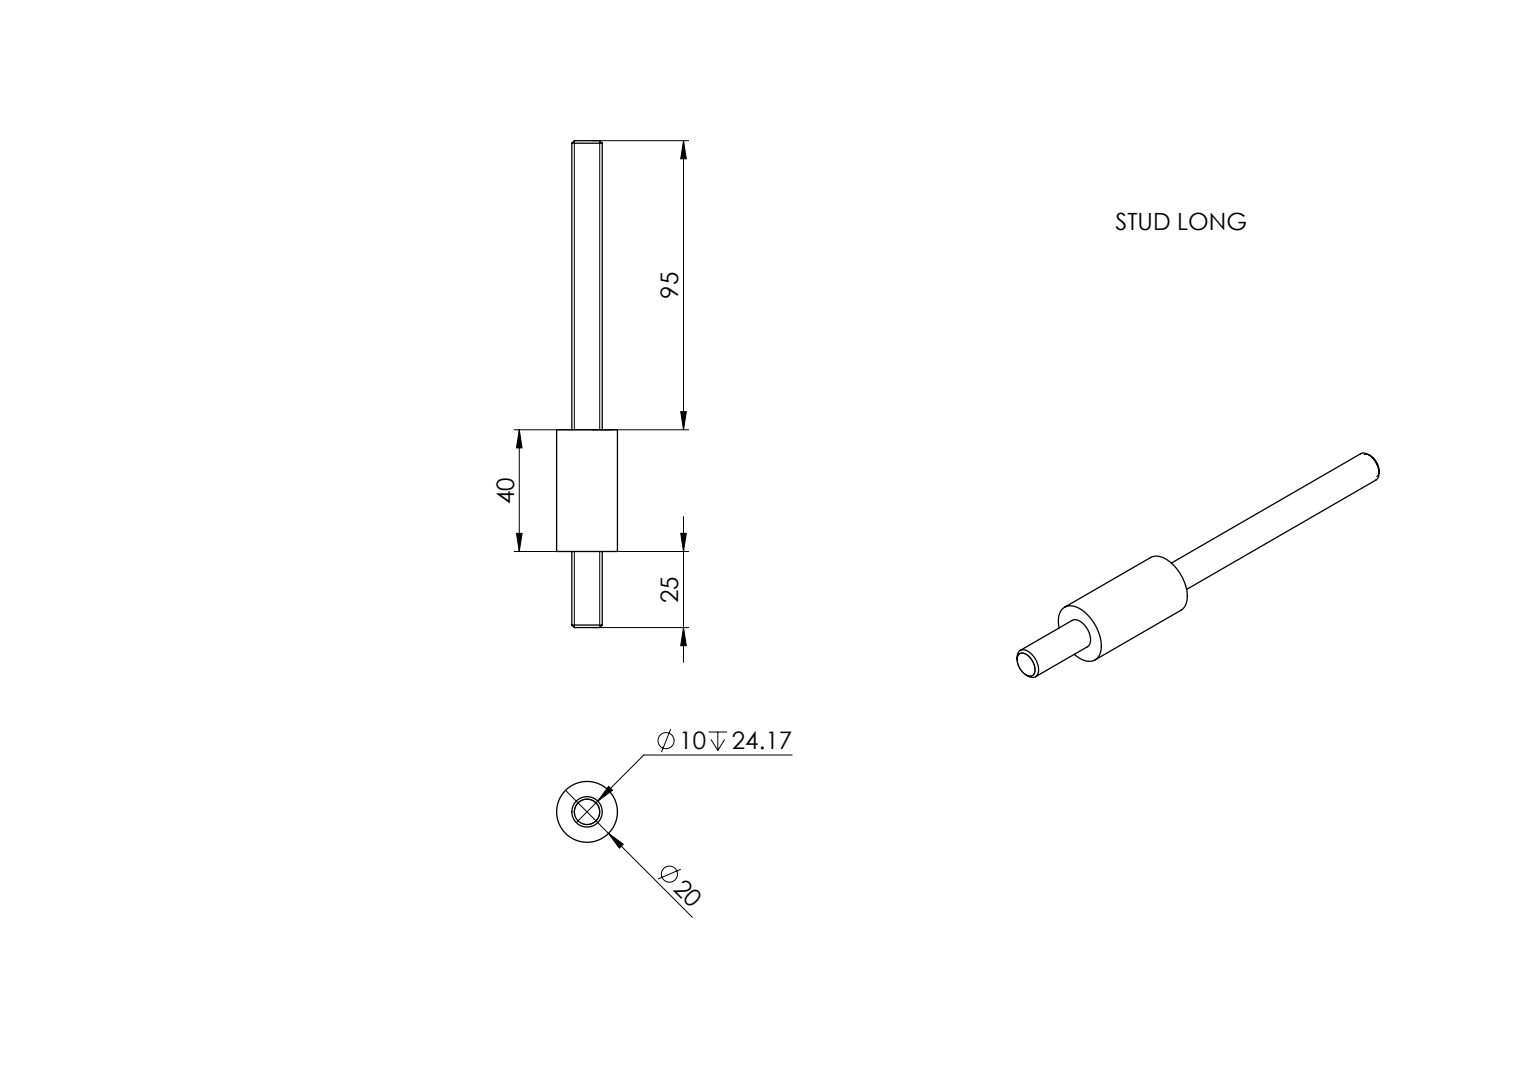
ISO-10303-21;
HEADER;
FILE_DESCRIPTION (('STEP AP214'),
    '1' );
FILE_NAME ('stud long.step',
    '2026-10-23T05:12:30',
    ( '' ),
    ( '' ),
    'SwSTEP 2.0',
    'SolidWorks 2026',
    '' );
FILE_SCHEMA (( 'AUTOMOTIVE_DESIGN' ));
ENDSEC;

DATA;
#5=CARTESIAN_POINT ( 'NONE',  ( -63.76644452187071721, 49.96174644486006855, -40.00000000000000000 ) ) ;
#28=CARTESIAN_POINT ( 'NONE',  ( -58.76644452187068168, 49.96174644486002592, -40.00000000000000000 ) ) ;
#77=DIRECTION ( 'NONE',  ( -0.000000000000000000, -0.000000000000000000, 1.000000000000000000 ) ) ;
#101=DIRECTION ( 'NONE',  ( 0.000000000000000000, 0.000000000000000000, 1.000000000000000000 ) ) ;
#189=CYLINDRICAL_SURFACE ( 'NONE', #7328, 5.000000000000004441 ) ;
#212=DIRECTION ( 'NONE',  ( -0.000000000000000000, -0.000000000000000000, -1.000000000000000000 ) ) ;
#233=DIRECTION ( 'NONE',  ( -1.000000000000000000, 0.000000000000000000, 0.000000000000000000 ) ) ;
#243=LINE ( 'NONE', #4981, #3185 ) ;
#258=AXIS2_PLACEMENT_3D ( 'NONE', #3304, #337, #5703 ) ;
#262=CARTESIAN_POINT ( 'NONE',  ( -68.76644452187068168, 49.96174644486002592, 0.000000000000000000 ) ) ;
#282=CARTESIAN_POINT ( 'NONE',  ( -72.93844452187067873, 49.96174644486002592, 25.00000000000000000 ) ) ;
#290=AXIS2_PLACEMENT_3D ( 'NONE', #4924, #77, #3632 ) ;
#297=AXIS2_PLACEMENT_3D ( 'NONE', #3501, #3421, #499 ) ;
#302=PRODUCT_DEFINITION ( 'UNKNOWN', '', #6087, #1721 ) ;
#312=EDGE_CURVE ( 'NONE', #3677, #520, #3029, .T. ) ;
#316=EDGE_CURVE ( 'NONE', #3677, #1170, #2354, .T. ) ;
#318=CARTESIAN_POINT ( 'NONE',  ( -68.76644452187068168, 49.96174644486002592, 24.17200000000001125 ) ) ;
#320=CARTESIAN_POINT ( 'NONE',  ( -68.76644452187068168, 49.96174644486002592, 24.17200000000001125 ) ) ;
#337=DIRECTION ( 'NONE',  ( 0.000000000000000000, 0.000000000000000000, 1.000000000000000000 ) ) ;
#350=ORIENTED_EDGE ( 'NONE', *, *, #2657, .F. ) ;
#374=EDGE_LOOP ( 'NONE', ( #679, #6781, #2050, #5404 ) ) ;
#380=VERTEX_POINT ( 'NONE', #1396 ) ;
#392=CIRCLE ( 'NONE', #1408, 10.00000000000000178 ) ;
#409=ADVANCED_FACE ( 'NONE', ( #5620 ), #3809, .T. ) ;
#429=STYLED_ITEM('',(#7837),#5821);
#440=ORIENTED_EDGE ( 'NONE', *, *, #2302, .F. ) ;
#455=CARTESIAN_POINT ( 'NONE',  ( -68.76644452187068168, 49.96174644486002592, 0.000000000000000000 ) ) ;
#469=DIRECTION ( 'NONE',  ( 1.000000000000000000, 0.000000000000000000, 0.000000000000000000 ) ) ;
#499=DIRECTION ( 'NONE',  ( 1.000000000000000000, 0.000000000000000000, 0.000000000000000000 ) ) ;
#509=CARTESIAN_POINT ( 'NONE',  ( -68.76644452187072432, 49.96174644486006855, -134.1720000000000255 ) ) ;
#520=VERTEX_POINT ( 'NONE', #2940 ) ;
#533=ORIENTED_EDGE ( 'NONE', *, *, #7554, .T. ) ;
#550=AXIS2_PLACEMENT_3D ( 'NONE', #3748, #3669, #5598 ) ;
#553=EDGE_LOOP ( 'NONE', ( #2394, #4192, #566, #4577 ) ) ;
#561=ORIENTED_EDGE ( 'NONE', *, *, #5713, .F. ) ;
#566=ORIENTED_EDGE ( 'NONE', *, *, #3757, .F. ) ;
#574=( GEOMETRIC_REPRESENTATION_CONTEXT ( 3 ) GLOBAL_UNCERTAINTY_ASSIGNED_CONTEXT ( ( #5327 ) ) GLOBAL_UNIT_ASSIGNED_CONTEXT ( ( #4488, #1529, #2096 ) ) REPRESENTATION_CONTEXT ( 'NONE', 'WORKASPACE' ) );
#581=PLANE ( 'NONE',  #2500 ) ;
#679=ORIENTED_EDGE ( 'NONE', *, *, #312, .F. ) ;
#732=CARTESIAN_POINT ( 'NONE',  ( -63.76644452187073142, 49.96174644486006855, -134.1720000000000255 ) ) ;
#748=CARTESIAN_POINT ( 'NONE',  ( -64.59444452187072727, 49.96174644486006855, -135.0000000000000000 ) ) ;
#810=DIRECTION ( 'NONE',  ( 0.000000000000000000, 0.000000000000000000, 1.000000000000000000 ) ) ;
#814=AXIS2_PLACEMENT_3D ( 'NONE', #2399, #6019, #1158 ) ;
#815=MECHANICAL_DESIGN_GEOMETRIC_PRESENTATION_REPRESENTATION('',(#2840),#574);
#820=SURFACE_STYLE_USAGE ( .BOTH. , #4962 ) ;
#836=DIRECTION ( 'NONE',  ( -1.000000000000000000, 0.000000000000000000, 0.000000000000000000 ) ) ;
#856=AXIS2_PLACEMENT_3D ( 'NONE', #4623, #4027, #1625 ) ;
#860=ORIENTED_EDGE ( 'NONE', *, *, #2548, .F. ) ;
#891=FACE_OUTER_BOUND ( 'NONE', #5087, .T. ) ;
#903=CARTESIAN_POINT ( 'NONE',  ( -63.76644452187067458, 49.96174644486002592, 0.000000000000000000 ) ) ;
#909=DIRECTION ( 'NONE',  ( -0.000000000000000000, -0.000000000000000000, -1.000000000000000000 ) ) ;
#983=CIRCLE ( 'NONE', #7538, 5.000000000000004441 ) ;
#995=CARTESIAN_POINT ( 'NONE',  ( -68.76644452187068168, 49.96174644486002592, 0.000000000000000000 ) ) ;
#1040=ORIENTED_EDGE ( 'NONE', *, *, #1788, .T. ) ;
#1111=CIRCLE ( 'NONE', #7411, 10.00000000000000178 ) ;
#1158=DIRECTION ( 'NONE',  ( 1.000000000000000000, 0.000000000000000000, -0.000000000000000000 ) ) ;
#1165=FACE_OUTER_BOUND ( 'NONE', #7589, .T. ) ;
#1170=VERTEX_POINT ( 'NONE', #282 ) ;
#1177=DIRECTION ( 'NONE',  ( -0.000000000000000000, -0.000000000000000000, 1.000000000000000000 ) ) ;
#1186=MECHANICAL_DESIGN_GEOMETRIC_PRESENTATION_REPRESENTATION('',(#429),#6358);
#1212=VERTEX_POINT ( 'NONE', #4586 ) ;
#1227=ORIENTED_EDGE ( 'NONE', *, *, #6300, .F. ) ;
#1239=AXIS2_PLACEMENT_3D ( 'NONE', #4603, #2287, #7634 ) ;
#1301=CARTESIAN_POINT ( 'NONE',  ( 0.000000000000000000, 0.000000000000000000, 0.000000000000000000 ) ) ;
#1302=CARTESIAN_POINT ( 'NONE',  ( -73.76644452187071010, 49.96174644486006855, -134.1720000000000255 ) ) ;
#1303=AXIS2_PLACEMENT_3D ( 'NONE', #509, #1177, #469 ) ;
#1323=DIRECTION ( 'NONE',  ( 1.000000000000000000, 0.000000000000000000, 0.000000000000000000 ) ) ;
#1327=ORIENTED_EDGE ( 'NONE', *, *, #3741, .T. ) ;
#1356=DIRECTION ( 'NONE',  ( -0.000000000000000000, -0.000000000000000000, -1.000000000000000000 ) ) ;
#1396=CARTESIAN_POINT ( 'NONE',  ( -78.76644452187068168, 49.96174644486002592, -40.00000000000000000 ) ) ;
#1398=DIRECTION ( 'NONE',  ( 1.000000000000000000, 0.000000000000000000, 0.000000000000000000 ) ) ;
#1408=AXIS2_PLACEMENT_3D ( 'NONE', #7465, #6806, #4429 ) ;
#1457=DIRECTION ( 'NONE',  ( 1.000000000000000000, 0.000000000000000000, 0.000000000000000000 ) ) ;
#1460=LINE ( 'NONE', #3759, #6409 ) ;
#1478=DIRECTION ( 'NONE',  ( -1.000000000000000000, 0.000000000000000000, 0.000000000000000000 ) ) ;
#1492=ADVANCED_FACE ( 'NONE', ( #5234, #1165 ), #581, .T. ) ;
#1529=( NAMED_UNIT ( * ) PLANE_ANGLE_UNIT ( ) SI_UNIT ( $, .RADIAN. ) );
#1535=CARTESIAN_POINT ( 'NONE',  ( -68.76644452187068168, 49.96174644486002592, 25.00000000000000000 ) ) ;
#1557=CIRCLE ( 'NONE', #550, 4.999999999999990230 ) ;
#1623=CARTESIAN_POINT ( 'NONE',  ( -73.76644452187072432, 49.96174644486006855, -40.00000000000000000 ) ) ;
#1624=APPLICATION_CONTEXT ( 'automotive_design' ) ;
#1625=DIRECTION ( 'NONE',  ( -1.000000000000000000, 0.000000000000000000, 0.000000000000000000 ) ) ;
#1633=CIRCLE ( 'NONE', #5418, 5.000000000000004441 ) ;
#1647=CONICAL_SURFACE ( 'NONE', #4166, 4.999999999999990230, 0.7853981633974482790 ) ;
#1708=EDGE_LOOP ( 'NONE', ( #1900, #7024 ) ) ;
#1721=PRODUCT_DEFINITION_CONTEXT ( 'detailed design', #3243, 'design' ) ;
#1728=ADVANCED_FACE ( 'NONE', ( #5694 ), #5143, .T. ) ;
#1770=VECTOR ( 'NONE', #5434, 1000.000000000000000 ) ;
#1788=EDGE_CURVE ( 'NONE', #7134, #3642, #3372, .T. ) ;
#1816=ORIENTED_EDGE ( 'NONE', *, *, #1788, .F. ) ;
#1819=( NAMED_UNIT ( * ) PLANE_ANGLE_UNIT ( ) SI_UNIT ( $, .RADIAN. ) );
#1824=AXIS2_PLACEMENT_3D ( 'NONE', #5094, #2113, #6402 ) ;
#1846=DIRECTION ( 'NONE',  ( -1.000000000000000000, 0.000000000000000000, 0.000000000000000000 ) ) ;
#1900=ORIENTED_EDGE ( 'NONE', *, *, #3757, .T. ) ;
#1904=AXIS2_PLACEMENT_3D ( 'NONE', #1535, #5639, #233 ) ;
#1933=( LENGTH_UNIT ( ) NAMED_UNIT ( * ) SI_UNIT ( .MILLI., .METRE. ) );
#1939=ORIENTED_EDGE ( 'NONE', *, *, #3219, .F. ) ;
#1945=CIRCLE ( 'NONE', #290, 4.171999999999995268 ) ;
#2043=DIRECTION ( 'NONE',  ( 1.000000000000000000, 0.000000000000000000, 0.000000000000000000 ) ) ;
#2050=ORIENTED_EDGE ( 'NONE', *, *, #7020, .T. ) ;
#2083=CARTESIAN_POINT ( 'NONE',  ( -68.76644452187068168, 49.96174644486002592, 0.000000000000000000 ) ) ;
#2096=( NAMED_UNIT ( * ) SI_UNIT ( $, .STERADIAN. ) SOLID_ANGLE_UNIT ( ) );
#2113=DIRECTION ( 'NONE',  ( -0.000000000000000000, -0.000000000000000000, 1.000000000000000000 ) ) ;
#2115=EDGE_CURVE ( 'NONE', #1212, #520, #5890, .T. ) ;
#2197=DIRECTION ( 'NONE',  ( -0.000000000000000000, -0.000000000000000000, 1.000000000000000000 ) ) ;
#2287=DIRECTION ( 'NONE',  ( -0.000000000000000000, -0.000000000000000000, -1.000000000000000000 ) ) ;
#2302=EDGE_CURVE ( 'NONE', #3642, #5742, #7106, .T. ) ;
#2315=ORIENTED_EDGE ( 'NONE', *, *, #3741, .F. ) ;
#2316=EDGE_CURVE ( 'NONE', #520, #1212, #2385, .T. ) ;
#2349=DIRECTION ( 'NONE',  ( 0.000000000000000000, 0.000000000000000000, 1.000000000000000000 ) ) ;
#2353=ORIENTED_EDGE ( 'NONE', *, *, #3219, .T. ) ;
#2354=CIRCLE ( 'NONE', #7131, 4.171999999999995268 ) ;
#2375=ORIENTED_EDGE ( 'NONE', *, *, #4853, .T. ) ;
#2380=CARTESIAN_POINT ( 'NONE',  ( -68.76644452187068168, 49.96174644486002592, 24.17200000000001125 ) ) ;
#2385=CIRCLE ( 'NONE', #856, 4.999999999999990230 ) ;
#2394=ORIENTED_EDGE ( 'NONE', *, *, #5334, .T. ) ;
#2399=CARTESIAN_POINT ( 'NONE',  ( -64.59444452187068464, 49.96174644486002592, 25.00000000000000000 ) ) ;
#2442=CARTESIAN_POINT ( 'NONE',  ( -68.76644452187068168, 49.96174644486002592, 25.00000000000000000 ) ) ;
#2450=DIRECTION ( 'NONE',  ( -0.7071067811865504593, 0.000000000000000000, -0.7071067811865445751 ) ) ;
#2500=AXIS2_PLACEMENT_3D ( 'NONE', #455, #101, #6727 ) ;
#2502=FACE_OUTER_BOUND ( 'NONE', #4802, .T. ) ;
#2548=EDGE_CURVE ( 'NONE', #7134, #3827, #6046, .T. ) ;
#2558=CARTESIAN_POINT ( 'NONE',  ( -63.76644452187068879, 49.96174644486002592, 24.17200000000001125 ) ) ;
#2651=EDGE_CURVE ( 'NONE', #520, #6904, #3242, .T. ) ;
#2657=EDGE_CURVE ( 'NONE', #2748, #7510, #1460, .T. ) ;
#2675=DIRECTION ( 'NONE',  ( 1.000000000000000000, 0.000000000000000000, 0.000000000000000000 ) ) ;
#2686=CARTESIAN_POINT ( 'NONE',  ( -68.76644452187072432, 49.96174644486006855, -134.1720000000000255 ) ) ;
#2735=EDGE_CURVE ( 'NONE', #3827, #3377, #4763, .T. ) ;
#2748=VERTEX_POINT ( 'NONE', #28 ) ;
#2756=CARTESIAN_POINT ( 'NONE',  ( -73.76644452187066747, 49.96174644486002592, 0.000000000000000000 ) ) ;
#2840=STYLED_ITEM ( 'NONE', ( #4407 ), #5288 ) ;
#2845=CARTESIAN_POINT ( 'NONE',  ( -78.76644452187068168, 49.96174644486002592, 0.000000000000000000 ) ) ;
#2926=EDGE_LOOP ( 'NONE', ( #3358, #5126, #2353, #6416 ) ) ;
#2928=EDGE_CURVE ( 'NONE', #2748, #380, #7672, .T. ) ;
#2940=CARTESIAN_POINT ( 'NONE',  ( -63.76644452187068879, 49.96174644486002592, 24.17200000000001125 ) ) ;
#2976=EDGE_LOOP ( 'NONE', ( #4159, #533, #4065, #5337 ) ) ;
#3005=AXIS2_PLACEMENT_3D ( 'NONE', #320, #909, #836 ) ;
#3029=LINE ( 'NONE', #2558, #6307 ) ;
#3036=CARTESIAN_POINT ( 'NONE',  ( -73.76644452187072432, 49.96174644486006855, -40.00000000000000000 ) ) ;
#3070=VECTOR ( 'NONE', #2450, 1000.000000000000000 ) ;
#3125=ADVANCED_FACE ( 'NONE', ( #7684 ), #4530, .T. ) ;
#3143=EDGE_LOOP ( 'NONE', ( #4610, #6396, #3626, #440 ) ) ;
#3154=AXIS2_PLACEMENT_3D ( 'NONE', #2380, #4052, #5915 ) ;
#3185=VECTOR ( 'NONE', #3805, 1000.000000000000000 ) ;
#3219=EDGE_CURVE ( 'NONE', #1212, #3662, #3971, .T. ) ;
#3221=CLOSED_SHELL ( 'NONE', ( #4175, #3792, #5574, #3125, #409, #6690, #4140, #1492, #6157, #7493, #1728, #3602, #5232, #4864 ) ) ;
#3222=DIRECTION ( 'NONE',  ( 0.000000000000000000, 0.000000000000000000, 1.000000000000000000 ) ) ;
#3226=EDGE_CURVE ( 'NONE', #3377, #5317, #1633, .T. ) ;
#3242=LINE ( 'NONE', #5828, #4768 ) ;
#3243=APPLICATION_CONTEXT ( 'automotive_design' ) ;
#3252=ORIENTED_EDGE ( 'NONE', *, *, #2928, .F. ) ;
#3271=DIRECTION ( 'NONE',  ( -0.000000000000000000, -0.000000000000000000, 1.000000000000000000 ) ) ;
#3273=SHAPE_REPRESENTATION_RELATIONSHIP ( 'NONE' , 'NONE' ,  #7725, #5288 ) ;
#3281=DIRECTION ( 'NONE',  ( 0.000000000000000000, 0.000000000000000000, 1.000000000000000000 ) ) ;
#3304=CARTESIAN_POINT ( 'NONE',  ( -68.76644452187068168, 49.96174644486002592, -40.00000000000000000 ) ) ;
#3331=DIRECTION ( 'NONE',  ( 0.000000000000000000, 0.000000000000000000, 1.000000000000000000 ) ) ;
#3348=CYLINDRICAL_SURFACE ( 'NONE', #7601, 4.999999999999990230 ) ;
#3358=ORIENTED_EDGE ( 'NONE', *, *, #2651, .F. ) ;
#3372=CIRCLE ( 'NONE', #3631, 4.171999999999995268 ) ;
#3377=VERTEX_POINT ( 'NONE', #1623 ) ;
#3408=AXIS2_PLACEMENT_3D ( 'NONE', #748, #5485, #4928 ) ;
#3410=DIRECTION ( 'NONE',  ( -0.000000000000000000, -0.000000000000000000, -1.000000000000000000 ) ) ;
#3421=DIRECTION ( 'NONE',  ( 0.000000000000000000, 0.000000000000000000, 1.000000000000000000 ) ) ;
#3501=CARTESIAN_POINT ( 'NONE',  ( -68.76644452187068168, 49.96174644486002592, 0.000000000000000000 ) ) ;
#3601=CYLINDRICAL_SURFACE ( 'NONE', #5573, 10.00000000000000178 ) ;
#3602=ADVANCED_FACE ( 'NONE', ( #2502 ), #4377, .T. ) ;
#3626=ORIENTED_EDGE ( 'NONE', *, *, #5334, .F. ) ;
#3631=AXIS2_PLACEMENT_3D ( 'NONE', #7582, #2197, #1398 ) ;
#3632=DIRECTION ( 'NONE',  ( 1.000000000000000000, 0.000000000000000000, 0.000000000000000000 ) ) ;
#3642=VERTEX_POINT ( 'NONE', #7342 ) ;
#3662=VERTEX_POINT ( 'NONE', #5414 ) ;
#3669=DIRECTION ( 'NONE',  ( -0.000000000000000000, -0.000000000000000000, 1.000000000000000000 ) ) ;
#3677=VERTEX_POINT ( 'NONE', #5603 ) ;
#3717=DIRECTION ( 'NONE',  ( -0.7071067811865474617, 8.659560562354932858E-17, 0.7071067811865474617 ) ) ;
#3737=LINE ( 'NONE', #6032, #3070 ) ;
#3741=EDGE_CURVE ( 'NONE', #380, #5243, #4455, .T. ) ;
#3748=CARTESIAN_POINT ( 'NONE',  ( -68.76644452187072432, 49.96174644486006855, -134.1720000000000255 ) ) ;
#3750=EDGE_CURVE ( 'NONE', #1170, #3677, #6186, .T. ) ;
#3752=ORIENTED_EDGE ( 'NONE', *, *, #6300, .T. ) ;
#3757=EDGE_CURVE ( 'NONE', #5317, #3377, #6688, .T. ) ;
#3758=DIRECTION ( 'NONE',  ( 0.000000000000000000, 0.000000000000000000, 1.000000000000000000 ) ) ;
#3759=CARTESIAN_POINT ( 'NONE',  ( -58.76644452187068168, 49.96174644486002592, -40.00000000000000000 ) ) ;
#3792=ADVANCED_FACE ( 'NONE', ( #5755 ), #1647, .T. ) ;
#3805=DIRECTION ( 'NONE',  ( -0.000000000000000000, -0.000000000000000000, 1.000000000000000000 ) ) ;
#3809=CYLINDRICAL_SURFACE ( 'NONE', #4985, 10.00000000000000178 ) ;
#3827=VERTEX_POINT ( 'NONE', #5835 ) ;
#3853=CARTESIAN_POINT ( 'NONE',  ( -68.76644452187068168, 49.96174644486002592, -40.00000000000000000 ) ) ;
#3860=EDGE_LOOP ( 'NONE', ( #2315, #5636, #6119, #1227 ) ) ;
#3863=DIRECTION ( 'NONE',  ( -0.000000000000000000, -0.000000000000000000, 1.000000000000000000 ) ) ;
#3906=DIRECTION ( 'NONE',  ( -0.000000000000000000, -0.000000000000000000, 1.000000000000000000 ) ) ;
#3918=DIRECTION ( 'NONE',  ( 1.000000000000000000, 0.000000000000000000, 0.000000000000000000 ) ) ;
#3944=DIRECTION ( 'NONE',  ( 1.000000000000000000, 0.000000000000000000, 0.000000000000000000 ) ) ;
#3971=LINE ( 'NONE', #2756, #5663 ) ;
#4003=VECTOR ( 'NONE', #7615, 1000.000000000000114 ) ;
#4008=CARTESIAN_POINT ( 'NONE',  ( -68.76644452187072432, 49.96174644486006855, -40.00000000000000000 ) ) ;
#4027=DIRECTION ( 'NONE',  ( -0.000000000000000000, -0.000000000000000000, -1.000000000000000000 ) ) ;
#4052=DIRECTION ( 'NONE',  ( -0.000000000000000000, -0.000000000000000000, -1.000000000000000000 ) ) ;
#4065=ORIENTED_EDGE ( 'NONE', *, *, #6397, .T. ) ;
#4074=CYLINDRICAL_SURFACE ( 'NONE', #6168, 5.000000000000004441 ) ;
#4131=ORIENTED_EDGE ( 'NONE', *, *, #4412, .T. ) ;
#4140=ADVANCED_FACE ( 'NONE', ( #6859, #891 ), #6899, .F. ) ;
#4159=ORIENTED_EDGE ( 'NONE', *, *, #2735, .F. ) ;
#4166=AXIS2_PLACEMENT_3D ( 'NONE', #2686, #6275, #3944 ) ;
#4175=ADVANCED_FACE ( 'NONE', ( #6784 ), #189, .T. ) ;
#4192=ORIENTED_EDGE ( 'NONE', *, *, #2735, .T. ) ;
#4202=CONICAL_SURFACE ( 'NONE', #1303, 4.999999999999990230, 0.7853981633974482790 ) ;
#4207=CIRCLE ( 'NONE', #297, 10.00000000000000178 ) ;
#4290=EDGE_LOOP ( 'NONE', ( #860, #1040, #5043, #4804 ) ) ;
#4377=PLANE ( 'NONE',  #3408 ) ;
#4407=PRESENTATION_STYLE_ASSIGNMENT (( #820 ) ) ;
#4412=EDGE_CURVE ( 'NONE', #3662, #6904, #5017, .T. ) ;
#4429=DIRECTION ( 'NONE',  ( 1.000000000000000000, 0.000000000000000000, 0.000000000000000000 ) ) ;
#4455=LINE ( 'NONE', #6351, #5166 ) ;
#4473=CARTESIAN_POINT ( 'NONE',  ( -68.76644452187068168, 49.96174644486002592, -40.00000000000000000 ) ) ;
#4479=( LENGTH_UNIT ( ) NAMED_UNIT ( * ) SI_UNIT ( .MILLI., .METRE. ) );
#4488=( LENGTH_UNIT ( ) NAMED_UNIT ( * ) SI_UNIT ( .MILLI., .METRE. ) );
#4530=CONICAL_SURFACE ( 'NONE', #3154, 4.999999999999990230, 0.7853981633974524978 ) ;
#4557=ORIENTED_EDGE ( 'NONE', *, *, #2651, .T. ) ;
#4570=ORIENTED_EDGE ( 'NONE', *, *, #4412, .F. ) ;
#4571=EDGE_LOOP ( 'NONE', ( #4131, #2375 ) ) ;
#4577=ORIENTED_EDGE ( 'NONE', *, *, #6397, .F. ) ;
#4586=CARTESIAN_POINT ( 'NONE',  ( -73.76644452187066747, 49.96174644486002592, 24.17200000000001125 ) ) ;
#4603=CARTESIAN_POINT ( 'NONE',  ( -68.76644452187068168, 49.96174644486002592, 0.000000000000000000 ) ) ;
#4610=ORIENTED_EDGE ( 'NONE', *, *, #5473, .T. ) ;
#4620=EDGE_CURVE ( 'NONE', #380, #2748, #1111, .T. ) ;
#4623=CARTESIAN_POINT ( 'NONE',  ( -68.76644452187068168, 49.96174644486002592, 24.17200000000001125 ) ) ;
#4706=DIRECTION ( 'NONE',  ( 1.000000000000000000, 0.000000000000000000, 0.000000000000000000 ) ) ;
#4738=DIRECTION ( 'NONE',  ( 1.000000000000000000, 0.000000000000000000, 0.000000000000000000 ) ) ;
#4763=LINE ( 'NONE', #3036, #1770 ) ;
#4768=VECTOR ( 'NONE', #5642, 1000.000000000000000 ) ;
#4778=CARTESIAN_POINT ( 'NONE',  ( -68.76644452187068168, 49.96174644486002592, -40.00000000000000000 ) ) ;
#4802=EDGE_LOOP ( 'NONE', ( #7337, #1816 ) ) ;
#4804=ORIENTED_EDGE ( 'NONE', *, *, #7554, .F. ) ;
#4853=EDGE_CURVE ( 'NONE', #6904, #3662, #983, .T. ) ;
#4864=ADVANCED_FACE ( 'NONE', ( #7664 ), #4074, .T. ) ;
#4924=CARTESIAN_POINT ( 'NONE',  ( -68.76644452187072432, 49.96174644486006855, -135.0000000000000000 ) ) ;
#4928=DIRECTION ( 'NONE',  ( -1.000000000000000000, 0.000000000000000000, -0.000000000000000000 ) ) ;
#4962=SURFACE_SIDE_STYLE ('',( #5074 ) ) ;
#4981=CARTESIAN_POINT ( 'NONE',  ( -63.76644452187071721, 49.96174644486006855, -40.00000000000000000 ) ) ;
#4985=AXIS2_PLACEMENT_3D ( 'NONE', #4473, #3331, #3918 ) ;
#5017=CIRCLE ( 'NONE', #1239, 5.000000000000004441 ) ;
#5043=ORIENTED_EDGE ( 'NONE', *, *, #2302, .T. ) ;
#5074=SURFACE_STYLE_FILL_AREA ( #7482 ) ;
#5087=EDGE_LOOP ( 'NONE', ( #3252, #6918 ) ) ;
#5094=CARTESIAN_POINT ( 'NONE',  ( -68.76644452187072432, 49.96174644486006855, -134.1720000000000255 ) ) ;
#5126=ORIENTED_EDGE ( 'NONE', *, *, #2316, .T. ) ;
#5130=DIRECTION ( 'NONE',  ( -0.000000000000000000, -0.000000000000000000, -1.000000000000000000 ) ) ;
#5143=CYLINDRICAL_SURFACE ( 'NONE', #5756, 4.999999999999990230 ) ;
#5166=VECTOR ( 'NONE', #7415, 1000.000000000000000 ) ;
#5211=DIRECTION ( 'NONE',  ( -1.000000000000000000, 0.000000000000000000, 0.000000000000000000 ) ) ;
#5232=ADVANCED_FACE ( 'NONE', ( #5919 ), #4202, .T. ) ;
#5234=FACE_BOUND ( 'NONE', #4571, .T. ) ;
#5243=VERTEX_POINT ( 'NONE', #2845 ) ;
#5288=ADVANCED_BREP_SHAPE_REPRESENTATION ( '', ( #5821, #7485 ), #6239 ) ;
#5317=VERTEX_POINT ( 'NONE', #5 ) ;
#5327=UNCERTAINTY_MEASURE_WITH_UNIT (LENGTH_MEASURE( 1.000000000000000082E-05 ), #4488, 'distance_accuracy_value', 'NONE');
#5333=FACE_OUTER_BOUND ( 'NONE', #3860, .T. ) ;
#5334=EDGE_CURVE ( 'NONE', #5742, #3827, #1557, .T. ) ;
#5337=ORIENTED_EDGE ( 'NONE', *, *, #3226, .F. ) ;
#5404=ORIENTED_EDGE ( 'NONE', *, *, #2316, .F. ) ;
#5414=CARTESIAN_POINT ( 'NONE',  ( -73.76644452187068168, 49.96174644486002592, 0.000000000000000000 ) ) ;
#5418=AXIS2_PLACEMENT_3D ( 'NONE', #4008, #3863, #7518 ) ;
#5434=DIRECTION ( 'NONE',  ( -0.000000000000000000, -0.000000000000000000, 1.000000000000000000 ) ) ;
#5471=ORIENTED_EDGE ( 'NONE', *, *, #316, .F. ) ;
#5473=EDGE_CURVE ( 'NONE', #3642, #7134, #1945, .T. ) ;
#5485=DIRECTION ( 'NONE',  ( 0.000000000000000000, 0.000000000000000000, -1.000000000000000000 ) ) ;
#5518=ORIENTED_EDGE ( 'NONE', *, *, #312, .T. ) ;
#5573=AXIS2_PLACEMENT_3D ( 'NONE', #4778, #2349, #4738 ) ;
#5574=ADVANCED_FACE ( 'NONE', ( #6232 ), #3348, .T. ) ;
#5598=DIRECTION ( 'NONE',  ( 1.000000000000000000, 0.000000000000000000, 0.000000000000000000 ) ) ;
#5603=CARTESIAN_POINT ( 'NONE',  ( -64.59444452187068464, 49.96174644486002592, 25.00000000000000000 ) ) ;
#5620=FACE_OUTER_BOUND ( 'NONE', #6386, .T. ) ;
#5636=ORIENTED_EDGE ( 'NONE', *, *, #4620, .T. ) ;
#5639=DIRECTION ( 'NONE',  ( -0.000000000000000000, -0.000000000000000000, -1.000000000000000000 ) ) ;
#5642=DIRECTION ( 'NONE',  ( -0.000000000000000000, -0.000000000000000000, -1.000000000000000000 ) ) ;
#5645=VECTOR ( 'NONE', #3717, 1000.000000000000114 ) ;
#5663=VECTOR ( 'NONE', #5667, 1000.000000000000000 ) ;
#5667=DIRECTION ( 'NONE',  ( -0.000000000000000000, -0.000000000000000000, -1.000000000000000000 ) ) ;
#5677=CARTESIAN_POINT ( 'NONE',  ( -68.76644452187072432, 49.96174644486006855, -40.00000000000000000 ) ) ;
#5694=FACE_OUTER_BOUND ( 'NONE', #2926, .T. ) ;
#5703=DIRECTION ( 'NONE',  ( 1.000000000000000000, 0.000000000000000000, -0.000000000000000000 ) ) ;
#5713=EDGE_CURVE ( 'NONE', #7510, #5243, #4207, .T. ) ;
#5742=VERTEX_POINT ( 'NONE', #732 ) ;
#5749=DIRECTION ( 'NONE',  ( -0.000000000000000000, -0.000000000000000000, -1.000000000000000000 ) ) ;
#5755=FACE_OUTER_BOUND ( 'NONE', #3143, .T. ) ;
#5756=AXIS2_PLACEMENT_3D ( 'NONE', #2083, #212, #1478 ) ;
#5821=MANIFOLD_SOLID_BREP ( 'M10 Machine Threads Stud2', #3221 ) ;
#5828=CARTESIAN_POINT ( 'NONE',  ( -63.76644452187068879, 49.96174644486002592, 0.000000000000000000 ) ) ;
#5835=CARTESIAN_POINT ( 'NONE',  ( -73.76644452187071010, 49.96174644486006855, -134.1720000000000255 ) ) ;
#5890=CIRCLE ( 'NONE', #3005, 4.999999999999990230 ) ;
#5915=DIRECTION ( 'NONE',  ( -1.000000000000000000, 0.000000000000000000, 0.000000000000000000 ) ) ;
#5919=FACE_OUTER_BOUND ( 'NONE', #4290, .T. ) ;
#5948=ORIENTED_EDGE ( 'NONE', *, *, #3750, .F. ) ;
#5977=DIRECTION ( 'NONE',  ( 1.000000000000000000, 0.000000000000000000, 0.000000000000000000 ) ) ;
#6019=DIRECTION ( 'NONE',  ( 0.000000000000000000, 0.000000000000000000, 1.000000000000000000 ) ) ;
#6032=CARTESIAN_POINT ( 'NONE',  ( -73.76644452187066747, 49.96174644486002592, 24.17200000000001125 ) ) ;
#6046=LINE ( 'NONE', #1302, #5645 ) ;
#6077=( NAMED_UNIT ( * ) SI_UNIT ( $, .STERADIAN. ) SOLID_ANGLE_UNIT ( ) );
#6087=PRODUCT_DEFINITION_FORMATION_WITH_SPECIFIED_SOURCE ( 'ANY', '', #6750, .NOT_KNOWN. ) ;
#6096=EDGE_LOOP ( 'NONE', ( #7109, #5518, #6548, #7126 ) ) ;
#6102=CIRCLE ( 'NONE', #1824, 4.999999999999990230 ) ;
#6119=ORIENTED_EDGE ( 'NONE', *, *, #2657, .T. ) ;
#6157=ADVANCED_FACE ( 'NONE', ( #7319 ), #6650, .T. ) ;
#6158=EDGE_LOOP ( 'NONE', ( #5948, #5471 ) ) ;
#6168=AXIS2_PLACEMENT_3D ( 'NONE', #6485, #7705, #4706 ) ;
#6179=DIRECTION ( 'NONE',  ( 0.7071067811865504593, 8.659560562354968603E-17, -0.7071067811865445751 ) ) ;
#6186=CIRCLE ( 'NONE', #1904, 4.171999999999995268 ) ;
#6219=PRODUCT_CONTEXT ( 'NONE', #1624, 'mechanical' ) ;
#6221=CARTESIAN_POINT ( 'NONE',  ( -68.76644452187068168, 49.96174644486002592, -40.00000000000000000 ) ) ;
#6228=CONICAL_SURFACE ( 'NONE', #7602, 4.999999999999990230, 0.7853981633974524978 ) ;
#6232=FACE_OUTER_BOUND ( 'NONE', #6592, .T. ) ;
#6239=( GEOMETRIC_REPRESENTATION_CONTEXT ( 3 ) GLOBAL_UNCERTAINTY_ASSIGNED_CONTEXT ( ( #6514 ) ) GLOBAL_UNIT_ASSIGNED_CONTEXT ( ( #1933, #1819, #6077 ) ) REPRESENTATION_CONTEXT ( 'NONE', 'WORKASPACE' ) );
#6275=DIRECTION ( 'NONE',  ( -0.000000000000000000, -0.000000000000000000, 1.000000000000000000 ) ) ;
#6300=EDGE_CURVE ( 'NONE', #5243, #7510, #392, .T. ) ;
#6307=VECTOR ( 'NONE', #6179, 1000.000000000000000 ) ;
#6351=CARTESIAN_POINT ( 'NONE',  ( -78.76644452187068168, 49.96174644486002592, -40.00000000000000000 ) ) ;
#6358=( GEOMETRIC_REPRESENTATION_CONTEXT ( 3 ) GLOBAL_UNCERTAINTY_ASSIGNED_CONTEXT ( ( #7318 ) ) GLOBAL_UNIT_ASSIGNED_CONTEXT ( ( #4479, #6892, #6815 ) ) REPRESENTATION_CONTEXT ( 'NONE', 'WORKASPACE' ) );
#6362=CARTESIAN_POINT ( 'NONE',  ( -58.76644452187068168, 49.96174644486002592, 0.000000000000000000 ) ) ;
#6386=EDGE_LOOP ( 'NONE', ( #7080, #1327, #561, #350 ) ) ;
#6396=ORIENTED_EDGE ( 'NONE', *, *, #2548, .T. ) ;
#6397=EDGE_CURVE ( 'NONE', #5742, #5317, #243, .T. ) ;
#6402=DIRECTION ( 'NONE',  ( 1.000000000000000000, 0.000000000000000000, 0.000000000000000000 ) ) ;
#6409=VECTOR ( 'NONE', #3281, 1000.000000000000000 ) ;
#6416=ORIENTED_EDGE ( 'NONE', *, *, #4853, .F. ) ;
#6485=CARTESIAN_POINT ( 'NONE',  ( -68.76644452187072432, 49.96174644486006855, -40.00000000000000000 ) ) ;
#6514=UNCERTAINTY_MEASURE_WITH_UNIT (LENGTH_MEASURE( 1.000000000000000082E-05 ), #1933, 'distance_accuracy_value', 'NONE');
#6534=ORIENTED_EDGE ( 'NONE', *, *, #2115, .T. ) ;
#6548=ORIENTED_EDGE ( 'NONE', *, *, #2115, .F. ) ;
#6592=EDGE_LOOP ( 'NONE', ( #6534, #4557, #4570, #1939 ) ) ;
#6650=PLANE ( 'NONE',  #814 ) ;
#6688=CIRCLE ( 'NONE', #7563, 5.000000000000004441 ) ;
#6690=ADVANCED_FACE ( 'NONE', ( #5333 ), #3601, .T. ) ;
#6727=DIRECTION ( 'NONE',  ( 1.000000000000000000, 0.000000000000000000, -0.000000000000000000 ) ) ;
#6750=PRODUCT ( 'stud long', 'stud long', '', ( #6219 ) ) ;
#6781=ORIENTED_EDGE ( 'NONE', *, *, #316, .T. ) ;
#6784=FACE_OUTER_BOUND ( 'NONE', #553, .T. ) ;
#6805=AXIS2_PLACEMENT_3D ( 'NONE', #6221, #810, #1323 ) ;
#6806=DIRECTION ( 'NONE',  ( 0.000000000000000000, 0.000000000000000000, 1.000000000000000000 ) ) ;
#6815=( NAMED_UNIT ( * ) SI_UNIT ( $, .STERADIAN. ) SOLID_ANGLE_UNIT ( ) );
#6859=FACE_BOUND ( 'NONE', #1708, .T. ) ;
#6892=( NAMED_UNIT ( * ) PLANE_ANGLE_UNIT ( ) SI_UNIT ( $, .RADIAN. ) );
#6899=PLANE ( 'NONE',  #258 ) ;
#6904=VERTEX_POINT ( 'NONE', #903 ) ;
#6918=ORIENTED_EDGE ( 'NONE', *, *, #4620, .F. ) ;
#6989=COLOUR_RGB ( '',0.8941176470588234615, 0.8941176470588234615, 0.8941176470588234615 ) ;
#6992=CARTESIAN_POINT ( 'NONE',  ( -63.76644452187073142, 49.96174644486006855, -134.1720000000000255 ) ) ;
#7020=EDGE_CURVE ( 'NONE', #1170, #1212, #3737, .T. ) ;
#7024=ORIENTED_EDGE ( 'NONE', *, *, #3226, .T. ) ;
#7080=ORIENTED_EDGE ( 'NONE', *, *, #2928, .T. ) ;
#7106=LINE ( 'NONE', #6992, #4003 ) ;
#7109=ORIENTED_EDGE ( 'NONE', *, *, #3750, .T. ) ;
#7114=CARTESIAN_POINT ( 'NONE',  ( -72.93844452187072136, 49.96174644486006855, -135.0000000000000000 ) ) ;
#7126=ORIENTED_EDGE ( 'NONE', *, *, #7020, .F. ) ;
#7131=AXIS2_PLACEMENT_3D ( 'NONE', #2442, #1356, #1846 ) ;
#7134=VERTEX_POINT ( 'NONE', #7114 ) ;
#7252=ORIENTED_EDGE ( 'NONE', *, *, #5713, .T. ) ;
#7318=UNCERTAINTY_MEASURE_WITH_UNIT (LENGTH_MEASURE( 1.000000000000000082E-05 ), #4479, 'distance_accuracy_value', 'NONE');
#7319=FACE_OUTER_BOUND ( 'NONE', #6158, .T. ) ;
#7328=AXIS2_PLACEMENT_3D ( 'NONE', #7404, #3271, #2675 ) ;
#7337=ORIENTED_EDGE ( 'NONE', *, *, #5473, .F. ) ;
#7342=CARTESIAN_POINT ( 'NONE',  ( -64.59444452187072727, 49.96174644486006855, -135.0000000000000000 ) ) ;
#7404=CARTESIAN_POINT ( 'NONE',  ( -68.76644452187072432, 49.96174644486006855, -40.00000000000000000 ) ) ;
#7411=AXIS2_PLACEMENT_3D ( 'NONE', #3853, #3222, #2043 ) ;
#7415=DIRECTION ( 'NONE',  ( 0.000000000000000000, 0.000000000000000000, 1.000000000000000000 ) ) ;
#7435=PRODUCT_DEFINITION_SHAPE ( 'NONE', 'NONE',  #302 ) ;
#7445=FILL_AREA_STYLE_COLOUR ( '', #6989 ) ;
#7465=CARTESIAN_POINT ( 'NONE',  ( -68.76644452187068168, 49.96174644486002592, 0.000000000000000000 ) ) ;
#7472=SHAPE_DEFINITION_REPRESENTATION ( #7435, #7725 ) ;
#7482=FILL_AREA_STYLE ('',( #7445 ) ) ;
#7485=AXIS2_PLACEMENT_3D ( 'NONE', #1301, #3758, #5977 ) ;
#7493=ADVANCED_FACE ( 'NONE', ( #7572 ), #6228, .T. ) ;
#7510=VERTEX_POINT ( 'NONE', #6362 ) ;
#7518=DIRECTION ( 'NONE',  ( 1.000000000000000000, 0.000000000000000000, 0.000000000000000000 ) ) ;
#7519=DIRECTION ( 'NONE',  ( -1.000000000000000000, 0.000000000000000000, 0.000000000000000000 ) ) ;
#7538=AXIS2_PLACEMENT_3D ( 'NONE', #995, #3410, #7624 ) ;
#7554=EDGE_CURVE ( 'NONE', #3827, #5742, #6102, .T. ) ;
#7563=AXIS2_PLACEMENT_3D ( 'NONE', #5677, #3906, #1457 ) ;
#7572=FACE_OUTER_BOUND ( 'NONE', #374, .T. ) ;
#7582=CARTESIAN_POINT ( 'NONE',  ( -68.76644452187072432, 49.96174644486006855, -135.0000000000000000 ) ) ;
#7589=EDGE_LOOP ( 'NONE', ( #7252, #3752 ) ) ;
#7601=AXIS2_PLACEMENT_3D ( 'NONE', #262, #5749, #7519 ) ;
#7602=AXIS2_PLACEMENT_3D ( 'NONE', #318, #5130, #5211 ) ;
#7615=DIRECTION ( 'NONE',  ( 0.7071067811865474617, 0.000000000000000000, 0.7071067811865474617 ) ) ;
#7624=DIRECTION ( 'NONE',  ( -1.000000000000000000, 0.000000000000000000, 0.000000000000000000 ) ) ;
#7634=DIRECTION ( 'NONE',  ( -1.000000000000000000, 0.000000000000000000, 0.000000000000000000 ) ) ;
#7664=FACE_OUTER_BOUND ( 'NONE', #2976, .T. ) ;
#7672=CIRCLE ( 'NONE', #6805, 10.00000000000000178 ) ;
#7684=FACE_OUTER_BOUND ( 'NONE', #6096, .T. ) ;
#7705=DIRECTION ( 'NONE',  ( -0.000000000000000000, -0.000000000000000000, 1.000000000000000000 ) ) ;
#7725=SHAPE_REPRESENTATION ( 'stud long', ( #7485 ), #6239 ) ;
#7831=COLOUR_RGB('Black',0.12,0.14,0.17);
#7832=FILL_AREA_STYLE_COLOUR('',#7831);
#7833=FILL_AREA_STYLE('',(#7832));
#7834=SURFACE_STYLE_FILL_AREA(#7833);
#7835=SURFACE_SIDE_STYLE('',(#7834));
#7836=SURFACE_STYLE_USAGE(.BOTH.,#7835);
#7837=PRESENTATION_STYLE_ASSIGNMENT((#7836));
ENDSEC;
END-ISO-10303-21;
